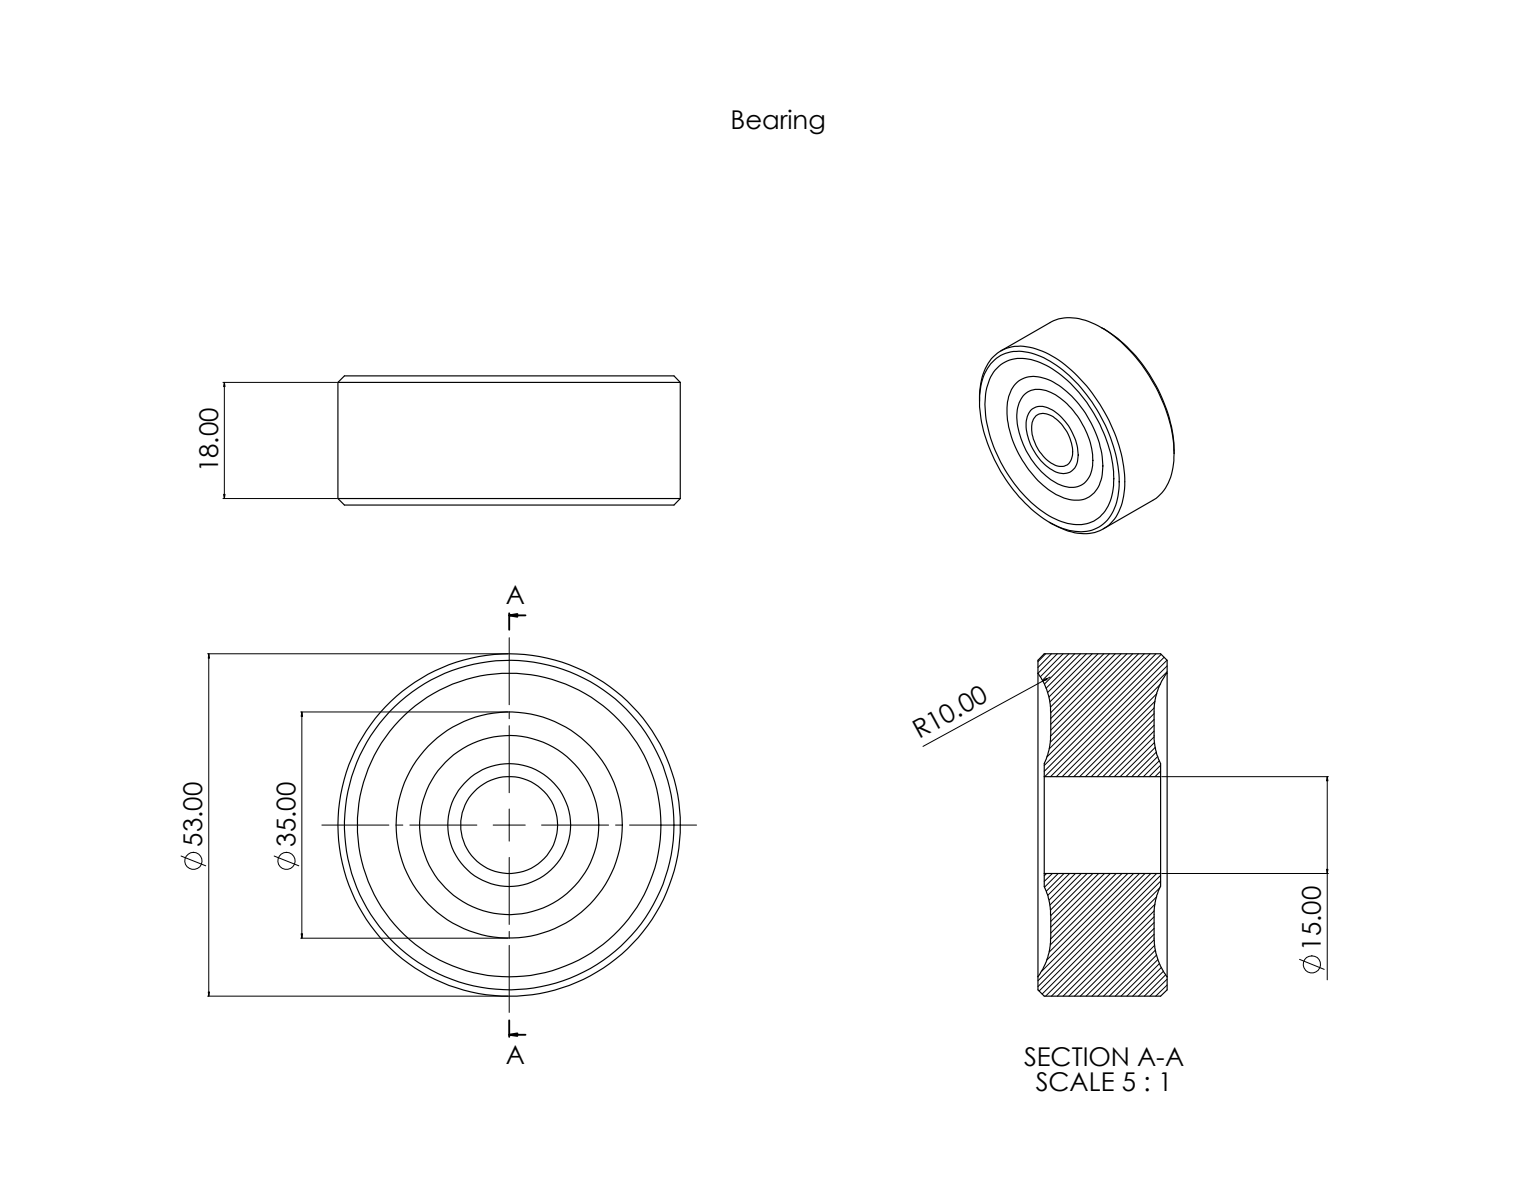
ISO-10303-21;
HEADER;
FILE_DESCRIPTION (('STEP AP214'),
    '1' );
FILE_NAME ('Bearing.step',
    '2026-10-19T17:36:30',
    ( '' ),
    ( '' ),
    'SwSTEP 2.0',
    'SolidWorks 2025',
    '' );
FILE_SCHEMA (( 'AUTOMOTIVE_DESIGN' ));
ENDSEC;

DATA;
#9=DIRECTION ( 'NONE',  ( -0.000000000000000000, -0.000000000000000000, -1.000000000000000000 ) ) ;
#14=DIRECTION ( 'NONE',  ( -0.000000000000000000, -0.000000000000000000, -1.000000000000000000 ) ) ;
#30=ORIENTED_EDGE ( 'NONE', *, *, #9025, .T. ) ;
#86=ADVANCED_FACE ( 'NONE', ( #9056 ), #3026, .F. ) ;
#151=CIRCLE ( 'NONE', #9264, 7.500000000000000000 ) ;
#175=EDGE_CURVE ( 'NONE', #10286, #4797, #4025, .T. ) ;
#182=DIRECTION ( 'NONE',  ( -0.7071067811865524577, 0.000000000000000000, -0.7071067811865426878 ) ) ;
#185=CONICAL_SURFACE ( 'NONE', #8085, 25.50000000000000711, 0.7853981633974552734 ) ;
#203=FACE_OUTER_BOUND ( 'NONE', #1468, .T. ) ;
#207=DIRECTION ( 'NONE',  ( 1.000000000000000000, 0.000000000000000000, 0.000000000000000000 ) ) ;
#209=DIRECTION ( 'NONE',  ( -0.000000000000000000, -0.000000000000000000, -1.000000000000000000 ) ) ;
#302=EDGE_CURVE ( 'NONE', #1347, #9626, #5867, .T. ) ;
#312=CIRCLE ( 'NONE', #4165, 9.499999999999994671 ) ;
#343=ADVANCED_FACE ( 'NONE', ( #7768 ), #9322, .F. ) ;
#362=( LENGTH_UNIT ( ) NAMED_UNIT ( * ) SI_UNIT ( .MILLI., .METRE. ) );
#374=CARTESIAN_POINT ( 'NONE',  ( 1.999999999999988010, 20.00000000000000355, 189.9999999999999716 ) ) ;
#386=DIRECTION ( 'NONE',  ( 0.000000000000000000, 0.000000000000000000, -1.000000000000000000 ) ) ;
#473=FACE_OUTER_BOUND ( 'NONE', #1842, .T. ) ;
#475=EDGE_CURVE ( 'NONE', #7179, #1407, #4444, .T. ) ;
#481=VERTEX_POINT ( 'NONE', #7503 ) ;
#524=DIRECTION ( 'NONE',  ( 1.000000000000000000, 0.000000000000000000, 0.000000000000000000 ) ) ;
#536=CARTESIAN_POINT ( 'NONE',  ( 27.49999999999999645, 20.00000000000000355, 189.9999999999999716 ) ) ;
#546=ADVANCED_FACE ( 'NONE', ( #3566 ), #11187, .T. ) ;
#568=CARTESIAN_POINT ( 'NONE',  ( 27.49999999999999645, 20.00000000000000355, 162.0000000000000000 ) ) ;
#631=DIRECTION ( 'NONE',  ( -0.000000000000000000, -0.000000000000000000, 1.000000000000000000 ) ) ;
#669=ORIENTED_EDGE ( 'NONE', *, *, #11328, .T. ) ;
#694=CARTESIAN_POINT ( 'NONE',  ( 27.49999999999999645, 20.00000000000000355, 189.9999999999999716 ) ) ;
#730=VERTEX_POINT ( 'NONE', #1726 ) ;
#754=DIRECTION ( 'NONE',  ( -0.000000000000000000, -0.000000000000000000, -1.000000000000000000 ) ) ;
#783=DIRECTION ( 'NONE',  ( 1.000000000000000000, 0.000000000000000000, 0.000000000000000000 ) ) ;
#792=ORIENTED_EDGE ( 'NONE', *, *, #1167, .F. ) ;
#818=CIRCLE ( 'NONE', #2648, 10.00000000000000000 ) ;
#833=EDGE_CURVE ( 'NONE', #4576, #10817, #6859, .T. ) ;
#847=EDGE_LOOP ( 'NONE', ( #1862, #12124, #11567, #792 ) ) ;
#851=CARTESIAN_POINT ( 'NONE',  ( 27.49999999999999645, 20.00000000000000355, 171.0000000000000000 ) ) ;
#856=CARTESIAN_POINT ( 'NONE',  ( 4.000000000000019540, 20.00000000000000711, 170.0000000000000000 ) ) ;
#861=DIRECTION ( 'NONE',  ( 1.000000000000000000, 0.000000000000000000, 0.000000000000000000 ) ) ;
#870=AXIS2_PLACEMENT_3D ( 'NONE', #1149, #3864, #4051 ) ;
#871=CARTESIAN_POINT ( 'NONE',  ( 1.000000000000000888, 20.00000000000000355, 170.9999999999999716 ) ) ;
#919=EDGE_CURVE ( 'NONE', #6911, #10286, #8230, .T. ) ;
#942=CARTESIAN_POINT ( 'NONE',  ( 41.35889894354065177, 20.00000000000000355, 162.0000000000000000 ) ) ;
#953=PRODUCT_CONTEXT ( 'NONE', #7801, 'mechanical' ) ;
#970=FACE_OUTER_BOUND ( 'NONE', #11386, .T. ) ;
#986=DIRECTION ( 'NONE',  ( 1.000000000000000000, 0.000000000000000000, 0.000000000000000000 ) ) ;
#998=DIRECTION ( 'NONE',  ( -0.000000000000000000, -0.000000000000000000, -1.000000000000000000 ) ) ;
#1040=FACE_OUTER_BOUND ( 'NONE', #4242, .T. ) ;
#1056=FACE_OUTER_BOUND ( 'NONE', #10210, .T. ) ;
#1061=ORIENTED_EDGE ( 'NONE', *, *, #10505, .T. ) ;
#1070=EDGE_CURVE ( 'NONE', #10817, #1347, #4044, .T. ) ;
#1075=AXIS2_PLACEMENT_3D ( 'NONE', #9726, #10725, #10926 ) ;
#1082=CIRCLE ( 'NONE', #11409, 17.49999999999996803 ) ;
#1094=AXIS2_PLACEMENT_3D ( 'NONE', #536, #2312, #8215 ) ;
#1097=CARTESIAN_POINT ( 'NONE',  ( 27.49999999999999645, 20.00000000000000355, 189.9999999999999716 ) ) ;
#1104=DIRECTION ( 'NONE',  ( 1.224646799147353207E-16, 1.000000000000000000, -0.000000000000000000 ) ) ;
#1122=CARTESIAN_POINT ( 'NONE',  ( 27.49999999999999645, 20.00000000000000355, 172.0000000000000000 ) ) ;
#1149=CARTESIAN_POINT ( 'NONE',  ( 27.49999999999999645, 20.00000000000000355, 189.9999999999999716 ) ) ;
#1157=FACE_OUTER_BOUND ( 'NONE', #5042, .T. ) ;
#1164=CARTESIAN_POINT ( 'NONE',  ( 19.99999999999999645, 20.00000000000000355, 189.9999999999999716 ) ) ;
#1167=EDGE_CURVE ( 'NONE', #1407, #9685, #1532, .T. ) ;
#1182=DIRECTION ( 'NONE',  ( 0.000000000000000000, 0.000000000000000000, -1.000000000000000000 ) ) ;
#1193=FACE_BOUND ( 'NONE', #3685, .T. ) ;
#1209=CARTESIAN_POINT ( 'NONE',  ( 27.49999999999999645, 20.00000000000000355, 189.9999999999999716 ) ) ;
#1211=AXIS2_PLACEMENT_3D ( 'NONE', #3932, #10461, #4763 ) ;
#1250=ORIENTED_EDGE ( 'NONE', *, *, #11960, .T. ) ;
#1305=CIRCLE ( 'NONE', #4943, 26.49999999999999645 ) ;
#1310=CARTESIAN_POINT ( 'NONE',  ( 27.49999999999999645, 20.00000000000000355, 170.0000000000000000 ) ) ;
#1318=AXIS2_PLACEMENT_3D ( 'NONE', #6837, #7793, #11665 ) ;
#1347=VERTEX_POINT ( 'NONE', #2706 ) ;
#1349=CARTESIAN_POINT ( 'NONE',  ( 27.49999999999999645, 20.00000000000000355, 197.9999999999999716 ) ) ;
#1369=AXIS2_PLACEMENT_3D ( 'NONE', #9446, #1818, #6703 ) ;
#1407=VERTEX_POINT ( 'NONE', #5698 ) ;
#1429=CARTESIAN_POINT ( 'NONE',  ( 34.99999999999999289, 20.00000000000000355, 171.0000000000000000 ) ) ;
#1446=TOROIDAL_SURFACE ( 'NONE', #12378, 13.85889894354065355, 10.00000000000000000 ) ;
#1468=EDGE_LOOP ( 'NONE', ( #3196, #7902 ) ) ;
#1499=AXIS2_PLACEMENT_3D ( 'NONE', #12513, #9480, #8642 ) ;
#1532=CIRCLE ( 'NONE', #6197, 10.00000000000000888 ) ;
#1544=ORIENTED_EDGE ( 'NONE', *, *, #11378, .T. ) ;
#1553=EDGE_CURVE ( 'NONE', #6911, #6345, #11267, .T. ) ;
#1584=AXIS2_PLACEMENT_3D ( 'NONE', #1209, #6901, #8873 ) ;
#1586=DIRECTION ( 'NONE',  ( 1.224646799147353207E-16, 1.000000000000000000, 0.000000000000000000 ) ) ;
#1598=EDGE_LOOP ( 'NONE', ( #3810, #5059 ) ) ;
#1620=DIRECTION ( 'NONE',  ( -0.000000000000000000, -0.000000000000000000, 1.000000000000000000 ) ) ;
#1675=PLANE ( 'NONE',  #2938 ) ;
#1700=CIRCLE ( 'NONE', #11843, 9.499999999999994671 ) ;
#1702=LINE ( 'NONE', #374, #11227 ) ;
#1726=CARTESIAN_POINT ( 'NONE',  ( 2.000000000000008882, 20.00000000000000711, 169.9999999999999716 ) ) ;
#1750=ORIENTED_EDGE ( 'NONE', *, *, #4293, .F. ) ;
#1791=EDGE_CURVE ( 'NONE', #8970, #4148, #8893, .T. ) ;
#1794=ORIENTED_EDGE ( 'NONE', *, *, #9260, .T. ) ;
#1818=DIRECTION ( 'NONE',  ( -0.000000000000000000, -0.000000000000000000, 1.000000000000000000 ) ) ;
#1821=FACE_OUTER_BOUND ( 'NONE', #2262, .T. ) ;
#1842=EDGE_LOOP ( 'NONE', ( #6785, #12387, #10361, #9801 ) ) ;
#1857=EDGE_CURVE ( 'NONE', #5215, #5293, #312, .T. ) ;
#1861=DIRECTION ( 'NONE',  ( 0.000000000000000000, 0.000000000000000000, -1.000000000000000000 ) ) ;
#1862=ORIENTED_EDGE ( 'NONE', *, *, #475, .F. ) ;
#1880=ADVANCED_FACE ( 'NONE', ( #8886, #203 ), #1675, .T. ) ;
#1893=AXIS2_PLACEMENT_3D ( 'NONE', #4279, #7320, #8219 ) ;
#1905=( NAMED_UNIT ( * ) SI_UNIT ( $, .STERADIAN. ) SOLID_ANGLE_UNIT ( ) );
#1926=DIRECTION ( 'NONE',  ( 0.000000000000000000, 0.000000000000000000, -1.000000000000000000 ) ) ;
#1928=VECTOR ( 'NONE', #3092, 1000.000000000000000 ) ;
#2003=TOROIDAL_SURFACE ( 'NONE', #3824, 13.85889894354065355, 10.00000000000000000 ) ;
#2075=AXIS2_PLACEMENT_3D ( 'NONE', #4841, #8707, #9787 ) ;
#2081=MANIFOLD_SOLID_BREP ( 'Fillet1', #9111 ) ;
#2093=DIRECTION ( 'NONE',  ( -0.000000000000000000, -0.000000000000000000, 1.000000000000000000 ) ) ;
#2098=DIRECTION ( 'NONE',  ( 1.000000000000000000, 0.000000000000000000, 0.000000000000000000 ) ) ;
#2107=CARTESIAN_POINT ( 'NONE',  ( 13.64110105645934290, 20.00000000000000355, 197.9999999999999716 ) ) ;
#2128=EDGE_LOOP ( 'NONE', ( #5597, #9875 ) ) ;
#2162=ORIENTED_EDGE ( 'NONE', *, *, #4585, .F. ) ;
#2167=DIRECTION ( 'NONE',  ( -0.000000000000000000, -0.000000000000000000, 1.000000000000000000 ) ) ;
#2177=VERTEX_POINT ( 'NONE', #10734 ) ;
#2208=CARTESIAN_POINT ( 'NONE',  ( 27.49999999999999645, 20.00000000000000355, 171.0000000000000000 ) ) ;
#2246=ORIENTED_EDGE ( 'NONE', *, *, #9611, .T. ) ;
#2262=EDGE_LOOP ( 'NONE', ( #5500, #669, #9036, #8194 ) ) ;
#2290=EDGE_LOOP ( 'NONE', ( #1544, #10095, #11839, #11489 ) ) ;
#2312=DIRECTION ( 'NONE',  ( 0.000000000000000000, 0.000000000000000000, -1.000000000000000000 ) ) ;
#2326=ORIENTED_EDGE ( 'NONE', *, *, #175, .F. ) ;
#2339=EDGE_LOOP ( 'NONE', ( #10440, #5022, #6178, #7639 ) ) ;
#2370=CARTESIAN_POINT ( 'NONE',  ( 18.00000000000000355, 20.00000000000000355, 171.0000000000000000 ) ) ;
#2372=DIRECTION ( 'NONE',  ( 1.000000000000000000, 0.000000000000000000, 0.000000000000000000 ) ) ;
#2373=CARTESIAN_POINT ( 'NONE',  ( 27.49999999999999645, 20.00000000000000355, 187.9999999999999716 ) ) ;
#2396=MECHANICAL_DESIGN_GEOMETRIC_PRESENTATION_REPRESENTATION('',(#6254),#7120);
#2404=FACE_BOUND ( 'NONE', #9472, .T. ) ;
#2443=AXIS2_PLACEMENT_3D ( 'NONE', #694, #12429, #4438 ) ;
#2520=AXIS2_PLACEMENT_3D ( 'NONE', #3090, #6958, #7856 ) ;
#2563=( NAMED_UNIT ( * ) SI_UNIT ( $, .STERADIAN. ) SOLID_ANGLE_UNIT ( ) );
#2576=ADVANCED_FACE ( 'NONE', ( #1157 ), #11345, .T. ) ;
#2634=AXIS2_PLACEMENT_3D ( 'NONE', #10717, #9844, #3935 ) ;
#2648=AXIS2_PLACEMENT_3D ( 'NONE', #9333, #1586, #12304 ) ;
#2706=CARTESIAN_POINT ( 'NONE',  ( 53.99999999999999289, 20.00000000000000711, 170.9999999999999716 ) ) ;
#2711=ORIENTED_EDGE ( 'NONE', *, *, #10237, .F. ) ;
#2715=CIRCLE ( 'NONE', #9816, 10.00000000000000888 ) ;
#2716=ADVANCED_FACE ( 'NONE', ( #4894 ), #4661, .F. ) ;
#2718=DIRECTION ( 'NONE',  ( 0.000000000000000000, 0.000000000000000000, -1.000000000000000000 ) ) ;
#2744=DIRECTION ( 'NONE',  ( 0.000000000000000000, 0.000000000000000000, 1.000000000000000000 ) ) ;
#2753=AXIS2_PLACEMENT_3D ( 'NONE', #11728, #3032, #12487 ) ;
#2782=ORIENTED_EDGE ( 'NONE', *, *, #7225, .T. ) ;
#2827=EDGE_LOOP ( 'NONE', ( #6882, #3164, #12009, #4594 ) ) ;
#2865=ADVANCED_FACE ( 'NONE', ( #7545, #5527 ), #4500, .T. ) ;
#2902=DIRECTION ( 'NONE',  ( -1.000000000000000000, 0.000000000000000000, 0.000000000000000000 ) ) ;
#2926=CIRCLE ( 'NONE', #2520, 25.50000000000000711 ) ;
#2933=DIRECTION ( 'NONE',  ( 0.000000000000000000, 0.000000000000000000, -1.000000000000000000 ) ) ;
#2935=( GEOMETRIC_REPRESENTATION_CONTEXT ( 3 ) GLOBAL_UNCERTAINTY_ASSIGNED_CONTEXT ( ( #3151 ) ) GLOBAL_UNIT_ASSIGNED_CONTEXT ( ( #10721, #5851, #1905 ) ) REPRESENTATION_CONTEXT ( 'NONE', 'WORKASPACE' ) );
#2938=AXIS2_PLACEMENT_3D ( 'NONE', #851, #1861, #7939 ) ;
#2959=DIRECTION ( 'NONE',  ( -1.000000000000000000, 0.000000000000000000, 0.000000000000000000 ) ) ;
#2965=DIRECTION ( 'NONE',  ( -0.000000000000000000, -0.000000000000000000, 1.000000000000000000 ) ) ;
#3005=ORIENTED_EDGE ( 'NONE', *, *, #10572, .T. ) ;
#3025=EDGE_CURVE ( 'NONE', #7179, #481, #818, .T. ) ;
#3026=TOROIDAL_SURFACE ( 'NONE', #6652, 17.49999999999996803, 10.00000000000000000 ) ;
#3032=DIRECTION ( 'NONE',  ( 0.000000000000000000, 0.000000000000000000, 1.000000000000000000 ) ) ;
#3070=CARTESIAN_POINT ( 'NONE',  ( 27.49999999999999645, 20.00000000000000355, 197.9999999999999716 ) ) ;
#3076=DIRECTION ( 'NONE',  ( -1.000000000000000000, 0.000000000000000000, 0.000000000000000000 ) ) ;
#3090=CARTESIAN_POINT ( 'NONE',  ( 27.49999999999999645, 20.00000000000000355, 189.9999999999999716 ) ) ;
#3092=DIRECTION ( 'NONE',  ( -0.000000000000000000, -0.000000000000000000, -1.000000000000000000 ) ) ;
#3100=CARTESIAN_POINT ( 'NONE',  ( 13.64110105645934290, 20.00000000000000355, 187.9999999999999716 ) ) ;
#3118=LINE ( 'NONE', #1164, #8438 ) ;
#3143=CARTESIAN_POINT ( 'NONE',  ( 27.49999999999999645, 20.00000000000000355, 172.0000000000000000 ) ) ;
#3151=UNCERTAINTY_MEASURE_WITH_UNIT (LENGTH_MEASURE( 1.000000000000000082E-05 ), #10721, 'distance_accuracy_value', 'NONE');
#3164=ORIENTED_EDGE ( 'NONE', *, *, #5095, .T. ) ;
#3168=AXIS2_PLACEMENT_3D ( 'NONE', #3277, #4032, #10889 ) ;
#3196=ORIENTED_EDGE ( 'NONE', *, *, #11378, .F. ) ;
#3201=CIRCLE ( 'NONE', #12514, 25.49999999999998934 ) ;
#3212=DIRECTION ( 'NONE',  ( -1.000000000000000000, 0.000000000000000000, 0.000000000000000000 ) ) ;
#3235=AXIS2_PLACEMENT_3D ( 'NONE', #3070, #11824, #2372 ) ;
#3253=ORIENTED_EDGE ( 'NONE', *, *, #9260, .F. ) ;
#3258=DIRECTION ( 'NONE',  ( -0.000000000000000000, -0.000000000000000000, -1.000000000000000000 ) ) ;
#3265=FACE_OUTER_BOUND ( 'NONE', #6855, .T. ) ;
#3277=CARTESIAN_POINT ( 'NONE',  ( 45.00000000000000000, 20.00000000000000711, 197.9999999999999716 ) ) ;
#3281=EDGE_CURVE ( 'NONE', #10732, #8970, #9129, .T. ) ;
#3299=ORIENTED_EDGE ( 'NONE', *, *, #9336, .F. ) ;
#3345=DIRECTION ( 'NONE',  ( 0.000000000000000000, 0.000000000000000000, -1.000000000000000000 ) ) ;
#3346=ADVANCED_FACE ( 'NONE', ( #6452, #4548 ), #7403, .F. ) ;
#3381=FACE_OUTER_BOUND ( 'NONE', #5742, .T. ) ;
#3411=AXIS2_PLACEMENT_3D ( 'NONE', #1122, #4987, #3076 ) ;
#3448=DIRECTION ( 'NONE',  ( 0.000000000000000000, 0.000000000000000000, 1.000000000000000000 ) ) ;
#3450=DIRECTION ( 'NONE',  ( 1.000000000000000000, 0.000000000000000000, 0.000000000000000000 ) ) ;
#3458=ORIENTED_EDGE ( 'NONE', *, *, #7225, .F. ) ;
#3485=ORIENTED_EDGE ( 'NONE', *, *, #833, .F. ) ;
#3519=DIRECTION ( 'NONE',  ( 0.000000000000000000, -1.000000000000000000, 0.000000000000000000 ) ) ;
#3563=EDGE_CURVE ( 'NONE', #730, #7703, #11363, .T. ) ;
#3566=FACE_OUTER_BOUND ( 'NONE', #7971, .T. ) ;
#3571=AXIS2_PLACEMENT_3D ( 'NONE', #1097, #209, #4425 ) ;
#3577=VERTEX_POINT ( 'NONE', #2370 ) ;
#3616=ORIENTED_EDGE ( 'NONE', *, *, #12033, .F. ) ;
#3620=EDGE_CURVE ( 'NONE', #10817, #4738, #11985, .T. ) ;
#3638=CARTESIAN_POINT ( 'NONE',  ( 27.49999999999999645, 20.00000000000000355, 188.9999999999999716 ) ) ;
#3664=CARTESIAN_POINT ( 'NONE',  ( 36.99999999999999289, 20.00000000000000355, 188.9999999999999716 ) ) ;
#3685=EDGE_LOOP ( 'NONE', ( #4549, #30 ) ) ;
#3712=VECTOR ( 'NONE', #10492, 1000.000000000000114 ) ;
#3721=TOROIDAL_SURFACE ( 'NONE', #10818, 17.49999999999996803, 10.00000000000000000 ) ;
#3723=DIRECTION ( 'NONE',  ( -1.000000000000000000, 0.000000000000000000, 0.000000000000000000 ) ) ;
#3749=VECTOR ( 'NONE', #11748, 1000.000000000000000 ) ;
#3752=DIRECTION ( 'NONE',  ( -0.000000000000000000, -0.000000000000000000, -1.000000000000000000 ) ) ;
#3774=CARTESIAN_POINT ( 'NONE',  ( 50.99999999999999289, 20.00000000000000711, 189.9999999999999716 ) ) ;
#3810=ORIENTED_EDGE ( 'NONE', *, *, #7903, .T. ) ;
#3814=AXIS2_PLACEMENT_3D ( 'NONE', #2107, #1104, #5984 ) ;
#3824=AXIS2_PLACEMENT_3D ( 'NONE', #9746, #10883, #7840 ) ;
#3851=DIRECTION ( 'NONE',  ( -1.000000000000000000, 0.000000000000000000, 0.000000000000000000 ) ) ;
#3864=DIRECTION ( 'NONE',  ( 0.000000000000000000, 0.000000000000000000, 1.000000000000000000 ) ) ;
#3901=ORIENTED_EDGE ( 'NONE', *, *, #3563, .F. ) ;
#3917=PLANE ( 'NONE',  #1318 ) ;
#3923=ADVANCED_FACE ( 'NONE', ( #6163 ), #1446, .F. ) ;
#3932=CARTESIAN_POINT ( 'NONE',  ( 27.49999999999999645, 20.00000000000000355, 187.9999999999999716 ) ) ;
#3935=DIRECTION ( 'NONE',  ( 1.000000000000000000, 0.000000000000000000, 0.000000000000000000 ) ) ;
#3940=SHAPE_REPRESENTATION_RELATIONSHIP ( 'NONE' , 'NONE' ,  #10013, #4901 ) ;
#3958=DIRECTION ( 'NONE',  ( 0.000000000000000000, 0.000000000000000000, -1.000000000000000000 ) ) ;
#4025=CIRCLE ( 'NONE', #7680, 10.00000000000000888 ) ;
#4032=DIRECTION ( 'NONE',  ( -1.224646799147353207E-16, 1.000000000000000000, 0.000000000000000000 ) ) ;
#4044=LINE ( 'NONE', #9955, #1928 ) ;
#4051=DIRECTION ( 'NONE',  ( 1.000000000000000000, 0.000000000000000000, 0.000000000000000000 ) ) ;
#4142=AXIS2_PLACEMENT_3D ( 'NONE', #9560, #12533, #861 ) ;
#4148=VERTEX_POINT ( 'NONE', #8436 ) ;
#4164=EDGE_LOOP ( 'NONE', ( #1794, #4301 ) ) ;
#4165=AXIS2_PLACEMENT_3D ( 'NONE', #3638, #6617, #9845 ) ;
#4225=CIRCLE ( 'NONE', #1584, 25.50000000000000711 ) ;
#4242=EDGE_LOOP ( 'NONE', ( #1061, #9593, #2711, #3299 ) ) ;
#4279=CARTESIAN_POINT ( 'NONE',  ( 27.49999999999999645, 20.00000000000000355, 188.9999999999999716 ) ) ;
#4288=ORIENTED_EDGE ( 'NONE', *, *, #7758, .T. ) ;
#4293=EDGE_CURVE ( 'NONE', #4576, #2177, #4225, .T. ) ;
#4301=ORIENTED_EDGE ( 'NONE', *, *, #3563, .T. ) ;
#4316=DIRECTION ( 'NONE',  ( 0.000000000000000000, 0.000000000000000000, 1.000000000000000000 ) ) ;
#4341=VECTOR ( 'NONE', #3752, 1000.000000000000000 ) ;
#4374=DIRECTION ( 'NONE',  ( 1.000000000000000000, 0.000000000000000000, 0.000000000000000000 ) ) ;
#4410=AXIS2_PLACEMENT_3D ( 'NONE', #2373, #10940, #3450 ) ;
#4425=DIRECTION ( 'NONE',  ( -1.000000000000000000, 0.000000000000000000, 0.000000000000000000 ) ) ;
#4438=DIRECTION ( 'NONE',  ( 1.000000000000000000, 0.000000000000000000, -0.000000000000000000 ) ) ;
#4439=ORIENTED_EDGE ( 'NONE', *, *, #10182, .F. ) ;
#4444=CIRCLE ( 'NONE', #7080, 23.49999999999999289 ) ;
#4500=PLANE ( 'NONE',  #2443 ) ;
#4548=FACE_BOUND ( 'NONE', #2128, .T. ) ;
#4549=ORIENTED_EDGE ( 'NONE', *, *, #7622, .T. ) ;
#4558=CARTESIAN_POINT ( 'NONE',  ( 18.00000000000000355, 20.00000000000000355, 188.9999999999999716 ) ) ;
#4576=VERTEX_POINT ( 'NONE', #8787 ) ;
#4585=EDGE_CURVE ( 'NONE', #11119, #10746, #6848, .T. ) ;
#4587=DIRECTION ( 'NONE',  ( 0.000000000000000000, -1.000000000000000000, 0.000000000000000000 ) ) ;
#4594=ORIENTED_EDGE ( 'NONE', *, *, #7758, .F. ) ;
#4610=DIRECTION ( 'NONE',  ( 0.000000000000000000, 0.000000000000000000, 1.000000000000000000 ) ) ;
#4661=TOROIDAL_SURFACE ( 'NONE', #9531, 17.50000000000000355, 10.00000000000000000 ) ;
#4689=ORIENTED_EDGE ( 'NONE', *, *, #5994, .F. ) ;
#4723=DIRECTION ( 'NONE',  ( -0.000000000000000000, -0.000000000000000000, 1.000000000000000000 ) ) ;
#4738=VERTEX_POINT ( 'NONE', #10183 ) ;
#4763=DIRECTION ( 'NONE',  ( 1.000000000000000000, 0.000000000000000000, 0.000000000000000000 ) ) ;
#4797=VERTEX_POINT ( 'NONE', #8157 ) ;
#4806=CIRCLE ( 'NONE', #8050, 7.500000000000000000 ) ;
#4820=CONICAL_SURFACE ( 'NONE', #6439, 26.49999999999999645, 0.7853981633974517207 ) ;
#4833=CARTESIAN_POINT ( 'NONE',  ( 27.49999999999999645, 20.00000000000000355, 197.9999999999999716 ) ) ;
#4841=CARTESIAN_POINT ( 'NONE',  ( 27.49999999999999645, 20.00000000000000355, 172.0000000000000000 ) ) ;
#4868=ORIENTED_EDGE ( 'NONE', *, *, #1553, .T. ) ;
#4894=FACE_OUTER_BOUND ( 'NONE', #6222, .T. ) ;
#4901=ADVANCED_BREP_SHAPE_REPRESENTATION ( '', ( #2081, #9021 ), #2935 ) ;
#4918=DIRECTION ( 'NONE',  ( -1.000000000000000000, 0.000000000000000000, 0.000000000000000000 ) ) ;
#4943=AXIS2_PLACEMENT_3D ( 'NONE', #12527, #1926, #11578 ) ;
#4987=DIRECTION ( 'NONE',  ( -0.000000000000000000, -0.000000000000000000, 1.000000000000000000 ) ) ;
#4988=ORIENTED_EDGE ( 'NONE', *, *, #9025, .F. ) ;
#4995=ORIENTED_EDGE ( 'NONE', *, *, #4585, .T. ) ;
#5022=ORIENTED_EDGE ( 'NONE', *, *, #919, .T. ) ;
#5042=EDGE_LOOP ( 'NONE', ( #9489, #3253, #2782, #7875 ) ) ;
#5059=ORIENTED_EDGE ( 'NONE', *, *, #1857, .T. ) ;
#5073=DIRECTION ( 'NONE',  ( -0.000000000000000000, -0.000000000000000000, -1.000000000000000000 ) ) ;
#5095=EDGE_CURVE ( 'NONE', #5215, #8335, #9299, .T. ) ;
#5179=DIRECTION ( 'NONE',  ( -0.000000000000000000, -0.000000000000000000, 1.000000000000000000 ) ) ;
#5187=EDGE_LOOP ( 'NONE', ( #5513, #6283 ) ) ;
#5215=VERTEX_POINT ( 'NONE', #4558 ) ;
#5245=ADVANCED_FACE ( 'NONE', ( #12301 ), #185, .T. ) ;
#5258=CIRCLE ( 'NONE', #1211, 17.50000000000000000 ) ;
#5259=CARTESIAN_POINT ( 'NONE',  ( 34.99999999999999289, 20.00000000000000355, 189.9999999999999716 ) ) ;
#5261=AXIS2_PLACEMENT_3D ( 'NONE', #5821, #4723, #986 ) ;
#5293=VERTEX_POINT ( 'NONE', #3664 ) ;
#5332=CIRCLE ( 'NONE', #1075, 9.499999999999994671 ) ;
#5349=CIRCLE ( 'NONE', #1499, 13.85889894354065710 ) ;
#5373=CIRCLE ( 'NONE', #4142, 26.49999999999999645 ) ;
#5420=DIRECTION ( 'NONE',  ( -0.000000000000000000, -0.000000000000000000, 1.000000000000000000 ) ) ;
#5451=AXIS2_PLACEMENT_3D ( 'NONE', #6681, #2093, #11803 ) ;
#5499=AXIS2_PLACEMENT_3D ( 'NONE', #6392, #4610, #5572 ) ;
#5500=ORIENTED_EDGE ( 'NONE', *, *, #3281, .F. ) ;
#5513=ORIENTED_EDGE ( 'NONE', *, *, #12033, .T. ) ;
#5523=CARTESIAN_POINT ( 'NONE',  ( 45.00000000000000000, 20.00000000000000711, 187.9999999999999716 ) ) ;
#5527=FACE_BOUND ( 'NONE', #5645, .T. ) ;
#5572=DIRECTION ( 'NONE',  ( 1.000000000000000000, 0.000000000000000000, -0.000000000000000000 ) ) ;
#5580=DIRECTION ( 'NONE',  ( -1.000000000000000000, 0.000000000000000000, 0.000000000000000000 ) ) ;
#5597=ORIENTED_EDGE ( 'NONE', *, *, #5994, .T. ) ;
#5633=CARTESIAN_POINT ( 'NONE',  ( 27.49999999999999645, 20.00000000000000355, 172.0000000000000000 ) ) ;
#5645=EDGE_LOOP ( 'NONE', ( #8468, #9144 ) ) ;
#5698=CARTESIAN_POINT ( 'NONE',  ( 50.99999999999997868, 20.00000000000000355, 170.0000000000000000 ) ) ;
#5705=CARTESIAN_POINT ( 'NONE',  ( 34.99999999999999289, 20.00000000000000355, 188.9999999999999716 ) ) ;
#5742=EDGE_LOOP ( 'NONE', ( #7247, #11998 ) ) ;
#5782=ORIENTED_EDGE ( 'NONE', *, *, #7927, .F. ) ;
#5816=VERTEX_POINT ( 'NONE', #7526 ) ;
#5821=CARTESIAN_POINT ( 'NONE',  ( 27.49999999999999645, 20.00000000000000355, 170.9999999999999716 ) ) ;
#5835=SHAPE_DEFINITION_REPRESENTATION ( #10056, #10013 ) ;
#5839=ADVANCED_FACE ( 'NONE', ( #7713 ), #2003, .F. ) ;
#5851=( NAMED_UNIT ( * ) PLANE_ANGLE_UNIT ( ) SI_UNIT ( $, .RADIAN. ) );
#5867=CIRCLE ( 'NONE', #5261, 26.49999999999999645 ) ;
#5897=AXIS2_PLACEMENT_3D ( 'NONE', #8209, #3258, #11061 ) ;
#5942=EDGE_LOOP ( 'NONE', ( #11633, #8084, #4288, #4988 ) ) ;
#5984=DIRECTION ( 'NONE',  ( -1.000000000000000000, 0.000000000000000000, 0.000000000000000000 ) ) ;
#5994=EDGE_CURVE ( 'NONE', #1407, #7179, #9107, .T. ) ;
#6077=EDGE_CURVE ( 'NONE', #4797, #6345, #5258, .T. ) ;
#6132=ORIENTED_EDGE ( 'NONE', *, *, #1167, .T. ) ;
#6163=FACE_OUTER_BOUND ( 'NONE', #5942, .T. ) ;
#6165=AXIS2_PLACEMENT_3D ( 'NONE', #8779, #1182, #4918 ) ;
#6173=AXIS2_PLACEMENT_3D ( 'NONE', #7250, #3448, #7313 ) ;
#6178=ORIENTED_EDGE ( 'NONE', *, *, #175, .T. ) ;
#6197=AXIS2_PLACEMENT_3D ( 'NONE', #11340, #11273, #3345 ) ;
#6222=EDGE_LOOP ( 'NONE', ( #11236, #4868, #6358, #2326 ) ) ;
#6233=CIRCLE ( 'NONE', #4410, 13.85889894354065710 ) ;
#6254=STYLED_ITEM('',(#12584),#2081);
#6280=CARTESIAN_POINT ( 'NONE',  ( 27.49999999999999645, 20.00000000000000355, 172.0000000000000000 ) ) ;
#6283=ORIENTED_EDGE ( 'NONE', *, *, #4293, .T. ) ;
#6309=CARTESIAN_POINT ( 'NONE',  ( 27.49999999999999645, 20.00000000000000355, 189.9999999999999716 ) ) ;
#6321=DIRECTION ( 'NONE',  ( 1.000000000000000000, 0.000000000000000000, 0.000000000000000000 ) ) ;
#6341=FACE_OUTER_BOUND ( 'NONE', #847, .T. ) ;
#6345=VERTEX_POINT ( 'NONE', #5523 ) ;
#6358=ORIENTED_EDGE ( 'NONE', *, *, #6077, .F. ) ;
#6392=CARTESIAN_POINT ( 'NONE',  ( 27.49999999999999645, 20.00000000000000355, 169.9999999999999716 ) ) ;
#6439=AXIS2_PLACEMENT_3D ( 'NONE', #7693, #2167, #2098 ) ;
#6452=FACE_OUTER_BOUND ( 'NONE', #4164, .T. ) ;
#6485=CARTESIAN_POINT ( 'NONE',  ( 27.49999999999999645, 20.00000000000000355, 170.0000000000000000 ) ) ;
#6502=CARTESIAN_POINT ( 'NONE',  ( 53.99999999999999289, 20.00000000000000355, 170.9999999999999716 ) ) ;
#6551=AXIS2_PLACEMENT_3D ( 'NONE', #9813, #998, #3212 ) ;
#6610=CIRCLE ( 'NONE', #12096, 13.85889894354065355 ) ;
#6617=DIRECTION ( 'NONE',  ( 0.000000000000000000, 0.000000000000000000, 1.000000000000000000 ) ) ;
#6652=AXIS2_PLACEMENT_3D ( 'NONE', #9491, #1620, #6321 ) ;
#6681=CARTESIAN_POINT ( 'NONE',  ( 27.49999999999999645, 20.00000000000000355, 171.0000000000000000 ) ) ;
#6703=DIRECTION ( 'NONE',  ( 1.000000000000000000, 0.000000000000000000, 0.000000000000000000 ) ) ;
#6785=ORIENTED_EDGE ( 'NONE', *, *, #1070, .F. ) ;
#6792=ORIENTED_EDGE ( 'NONE', *, *, #8850, .T. ) ;
#6833=DIRECTION ( 'NONE',  ( -0.000000000000000000, -0.000000000000000000, 1.000000000000000000 ) ) ;
#6837=CARTESIAN_POINT ( 'NONE',  ( 27.49999999999999645, 20.00000000000000355, 188.9999999999999716 ) ) ;
#6848=CIRCLE ( 'NONE', #3411, 13.85889894354065355 ) ;
#6855=EDGE_LOOP ( 'NONE', ( #1750, #10407, #8775, #9220 ) ) ;
#6859=LINE ( 'NONE', #8958, #3749 ) ;
#6882=ORIENTED_EDGE ( 'NONE', *, *, #1857, .F. ) ;
#6901=DIRECTION ( 'NONE',  ( 0.000000000000000000, 0.000000000000000000, 1.000000000000000000 ) ) ;
#6911=VERTEX_POINT ( 'NONE', #3774 ) ;
#6918=DIRECTION ( 'NONE',  ( 1.000000000000000000, 0.000000000000000000, 0.000000000000000000 ) ) ;
#6958=DIRECTION ( 'NONE',  ( 0.000000000000000000, 0.000000000000000000, 1.000000000000000000 ) ) ;
#6986=CARTESIAN_POINT ( 'NONE',  ( 27.49999999999999645, 20.00000000000000355, 169.9999999999999716 ) ) ;
#6994=ADVANCED_FACE ( 'NONE', ( #8728 ), #12034, .F. ) ;
#6998=EDGE_CURVE ( 'NONE', #9685, #481, #1082, .T. ) ;
#7080=AXIS2_PLACEMENT_3D ( 'NONE', #6485, #5420, #9291 ) ;
#7120=( GEOMETRIC_REPRESENTATION_CONTEXT ( 3 ) GLOBAL_UNCERTAINTY_ASSIGNED_CONTEXT ( ( #11655 ) ) GLOBAL_UNIT_ASSIGNED_CONTEXT ( ( #362, #12213, #2563 ) ) REPRESENTATION_CONTEXT ( 'NONE', 'WORKASPACE' ) );
#7153=EDGE_CURVE ( 'NONE', #4738, #10817, #1305, .T. ) ;
#7160=FACE_OUTER_BOUND ( 'NONE', #12382, .T. ) ;
#7164=ORIENTED_EDGE ( 'NONE', *, *, #7927, .T. ) ;
#7179=VERTEX_POINT ( 'NONE', #856 ) ;
#7225=EDGE_CURVE ( 'NONE', #7703, #1347, #12345, .T. ) ;
#7247=ORIENTED_EDGE ( 'NONE', *, *, #6077, .T. ) ;
#7248=CARTESIAN_POINT ( 'NONE',  ( 27.49999999999999645, 20.00000000000000355, 189.0000000000000000 ) ) ;
#7250=CARTESIAN_POINT ( 'NONE',  ( 27.49999999999999645, 20.00000000000000355, 187.9999999999999716 ) ) ;
#7251=DIRECTION ( 'NONE',  ( -1.000000000000000000, 0.000000000000000000, 0.000000000000000000 ) ) ;
#7303=ADVANCED_FACE ( 'NONE', ( #1056 ), #9199, .F. ) ;
#7313=DIRECTION ( 'NONE',  ( 1.000000000000000000, 0.000000000000000000, -0.000000000000000000 ) ) ;
#7320=DIRECTION ( 'NONE',  ( 0.000000000000000000, 0.000000000000000000, 1.000000000000000000 ) ) ;
#7395=CARTESIAN_POINT ( 'NONE',  ( 13.64110105645934290, 20.00000000000000355, 162.0000000000000000 ) ) ;
#7403=PLANE ( 'NONE',  #5499 ) ;
#7440=DIRECTION ( 'NONE',  ( -0.000000000000000000, -0.000000000000000000, -1.000000000000000000 ) ) ;
#7472=DIRECTION ( 'NONE',  ( -1.224646799147353207E-16, 1.000000000000000000, 0.000000000000000000 ) ) ;
#7495=EDGE_LOOP ( 'NONE', ( #8435, #9099 ) ) ;
#7503=CARTESIAN_POINT ( 'NONE',  ( 10.00000000000003020, 20.00000000000000711, 172.0000000000000000 ) ) ;
#7525=CARTESIAN_POINT ( 'NONE',  ( 41.35889894354065177, 20.00000000000000355, 187.9999999999999716 ) ) ;
#7526=CARTESIAN_POINT ( 'NONE',  ( 19.99999999999999645, 20.00000000000000355, 188.9999999999999716 ) ) ;
#7544=ADVANCED_FACE ( 'NONE', ( #3265 ), #9805, .T. ) ;
#7545=FACE_OUTER_BOUND ( 'NONE', #5187, .T. ) ;
#7561=EDGE_LOOP ( 'NONE', ( #7625, #7788 ) ) ;
#7586=CIRCLE ( 'NONE', #1893, 7.500000000000000000 ) ;
#7601=AXIS2_PLACEMENT_3D ( 'NONE', #7395, #10541, #2933 ) ;
#7622=EDGE_CURVE ( 'NONE', #10986, #8335, #5349, .T. ) ;
#7625=ORIENTED_EDGE ( 'NONE', *, *, #10505, .F. ) ;
#7639=ORIENTED_EDGE ( 'NONE', *, *, #10029, .F. ) ;
#7680=AXIS2_PLACEMENT_3D ( 'NONE', #12217, #3519, #3958 ) ;
#7693=CARTESIAN_POINT ( 'NONE',  ( 27.49999999999999645, 20.00000000000000355, 170.9999999999999716 ) ) ;
#7696=DIRECTION ( 'NONE',  ( 0.000000000000000000, 0.000000000000000000, 1.000000000000000000 ) ) ;
#7703=VERTEX_POINT ( 'NONE', #10540 ) ;
#7713=FACE_OUTER_BOUND ( 'NONE', #2290, .T. ) ;
#7728=EDGE_CURVE ( 'NONE', #4738, #9626, #8581, .T. ) ;
#7732=CARTESIAN_POINT ( 'NONE',  ( 27.49999999999999645, 20.00000000000000355, 189.9999999999999716 ) ) ;
#7758=EDGE_CURVE ( 'NONE', #5293, #10986, #2715, .T. ) ;
#7768=FACE_OUTER_BOUND ( 'NONE', #2827, .T. ) ;
#7769=LINE ( 'NONE', #9740, #7853 ) ;
#7787=AXIS2_PLACEMENT_3D ( 'NONE', #7732, #754, #3723 ) ;
#7788=ORIENTED_EDGE ( 'NONE', *, *, #11328, .F. ) ;
#7793=DIRECTION ( 'NONE',  ( 0.000000000000000000, 0.000000000000000000, 1.000000000000000000 ) ) ;
#7801=APPLICATION_CONTEXT ( 'automotive_design' ) ;
#7821=CARTESIAN_POINT ( 'NONE',  ( 27.49999999999999645, 20.00000000000000355, 188.9999999999999716 ) ) ;
#7840=DIRECTION ( 'NONE',  ( -1.000000000000000000, 0.000000000000000000, 0.000000000000000000 ) ) ;
#7848=AXIS2_PLACEMENT_3D ( 'NONE', #942, #7472, #3851 ) ;
#7853=VECTOR ( 'NONE', #11641, 1000.000000000000114 ) ;
#7856=DIRECTION ( 'NONE',  ( 1.000000000000000000, 0.000000000000000000, 0.000000000000000000 ) ) ;
#7875=ORIENTED_EDGE ( 'NONE', *, *, #12257, .F. ) ;
#7902=ORIENTED_EDGE ( 'NONE', *, *, #10132, .F. ) ;
#7903=EDGE_CURVE ( 'NONE', #5293, #5215, #5332, .T. ) ;
#7927=EDGE_CURVE ( 'NONE', #481, #9685, #11607, .T. ) ;
#7939=DIRECTION ( 'NONE',  ( 1.000000000000000000, 0.000000000000000000, 0.000000000000000000 ) ) ;
#7971=EDGE_LOOP ( 'NONE', ( #11116, #10735, #8923, #9671 ) ) ;
#8021=ORIENTED_EDGE ( 'NONE', *, *, #3620, .F. ) ;
#8050=AXIS2_PLACEMENT_3D ( 'NONE', #7821, #7696, #8643 ) ;
#8052=APPLICATION_CONTEXT ( 'automotive_design' ) ;
#8084=ORIENTED_EDGE ( 'NONE', *, *, #7903, .F. ) ;
#8085=AXIS2_PLACEMENT_3D ( 'NONE', #8679, #2718, #5580 ) ;
#8105=AXIS2_PLACEMENT_3D ( 'NONE', #9355, #7440, #7251 ) ;
#8148=DIRECTION ( 'NONE',  ( 0.000000000000000000, 0.000000000000000000, -1.000000000000000000 ) ) ;
#8157=CARTESIAN_POINT ( 'NONE',  ( 9.999999999999991118, 20.00000000000000355, 187.9999999999999716 ) ) ;
#8194=ORIENTED_EDGE ( 'NONE', *, *, #1791, .F. ) ;
#8209=CARTESIAN_POINT ( 'NONE',  ( 27.49999999999999645, 20.00000000000000355, 169.9999999999999716 ) ) ;
#8214=CIRCLE ( 'NONE', #7601, 10.00000000000000888 ) ;
#8215=DIRECTION ( 'NONE',  ( -1.000000000000000000, 0.000000000000000000, 0.000000000000000000 ) ) ;
#8219=DIRECTION ( 'NONE',  ( 1.000000000000000000, 0.000000000000000000, 0.000000000000000000 ) ) ;
#8230=CIRCLE ( 'NONE', #2753, 23.49999999999999289 ) ;
#8303=ORIENTED_EDGE ( 'NONE', *, *, #6998, .T. ) ;
#8321=EDGE_CURVE ( 'NONE', #10286, #6911, #10388, .T. ) ;
#8335=VERTEX_POINT ( 'NONE', #3100 ) ;
#8415=ADVANCED_FACE ( 'NONE', ( #7160, #2404 ), #9202, .T. ) ;
#8426=DIRECTION ( 'NONE',  ( 0.000000000000000000, 0.000000000000000000, 1.000000000000000000 ) ) ;
#8435=ORIENTED_EDGE ( 'NONE', *, *, #10237, .T. ) ;
#8436=CARTESIAN_POINT ( 'NONE',  ( 19.99999999999999645, 20.00000000000000355, 171.0000000000000000 ) ) ;
#8438=VECTOR ( 'NONE', #14, 1000.000000000000000 ) ;
#8468=ORIENTED_EDGE ( 'NONE', *, *, #8321, .F. ) ;
#8517=VECTOR ( 'NONE', #5073, 1000.000000000000000 ) ;
#8581=LINE ( 'NONE', #9542, #4341 ) ;
#8642=DIRECTION ( 'NONE',  ( 1.000000000000000000, 0.000000000000000000, 0.000000000000000000 ) ) ;
#8643=DIRECTION ( 'NONE',  ( 1.000000000000000000, 0.000000000000000000, 0.000000000000000000 ) ) ;
#8679=CARTESIAN_POINT ( 'NONE',  ( 27.49999999999999645, 20.00000000000000355, 189.9999999999999716 ) ) ;
#8688=AXIS2_PLACEMENT_3D ( 'NONE', #1310, #5179, #524 ) ;
#8707=DIRECTION ( 'NONE',  ( 0.000000000000000000, 0.000000000000000000, -1.000000000000000000 ) ) ;
#8728=FACE_OUTER_BOUND ( 'NONE', #2339, .T. ) ;
#8740=FACE_BOUND ( 'NONE', #7561, .T. ) ;
#8755=DIRECTION ( 'NONE',  ( -1.000000000000000000, 0.000000000000000000, 0.000000000000000000 ) ) ;
#8775=ORIENTED_EDGE ( 'NONE', *, *, #7153, .F. ) ;
#8779=CARTESIAN_POINT ( 'NONE',  ( 27.49999999999999645, 20.00000000000000355, 162.0000000000000000 ) ) ;
#8787=CARTESIAN_POINT ( 'NONE',  ( 53.00000000000000711, 20.00000000000000711, 189.9999999999999716 ) ) ;
#8788=EDGE_LOOP ( 'NONE', ( #11491, #4689, #6132, #5782 ) ) ;
#8850=EDGE_CURVE ( 'NONE', #730, #9626, #7769, .T. ) ;
#8873=DIRECTION ( 'NONE',  ( 1.000000000000000000, 0.000000000000000000, 0.000000000000000000 ) ) ;
#8886=FACE_BOUND ( 'NONE', #7495, .T. ) ;
#8893=CIRCLE ( 'NONE', #5451, 7.500000000000000000 ) ;
#8915=ORIENTED_EDGE ( 'NONE', *, *, #10132, .T. ) ;
#8923=ORIENTED_EDGE ( 'NONE', *, *, #302, .T. ) ;
#8958=CARTESIAN_POINT ( 'NONE',  ( 53.00000000000000711, 20.00000000000000711, 189.9999999999999716 ) ) ;
#8970=VERTEX_POINT ( 'NONE', #1429 ) ;
#8974=ADVANCED_FACE ( 'NONE', ( #473 ), #11188, .T. ) ;
#9021=AXIS2_PLACEMENT_3D ( 'NONE', #11433, #2744, #207 ) ;
#9025=EDGE_CURVE ( 'NONE', #8335, #10986, #6233, .T. ) ;
#9036=ORIENTED_EDGE ( 'NONE', *, *, #9336, .T. ) ;
#9056=FACE_OUTER_BOUND ( 'NONE', #8788, .T. ) ;
#9099=ORIENTED_EDGE ( 'NONE', *, *, #1791, .T. ) ;
#9107=CIRCLE ( 'NONE', #8688, 23.49999999999999289 ) ;
#9111=CLOSED_SHELL ( 'NONE', ( #2716, #343, #5839, #11720, #7544, #9315, #546, #9382, #12380, #11846, #2865, #3346, #8974, #8415, #2576, #5245, #11947, #1880, #86, #7303, #3923, #6994 ) ) ;
#9129=LINE ( 'NONE', #5259, #8517 ) ;
#9144=ORIENTED_EDGE ( 'NONE', *, *, #919, .F. ) ;
#9145=AXIS2_PLACEMENT_3D ( 'NONE', #7248, #8148, #11121 ) ;
#9159=VERTEX_POINT ( 'NONE', #11246 ) ;
#9199=TOROIDAL_SURFACE ( 'NONE', #6165, 13.85889894354065355, 10.00000000000000000 ) ;
#9202=PLANE ( 'NONE',  #10583 ) ;
#9220=ORIENTED_EDGE ( 'NONE', *, *, #11960, .F. ) ;
#9230=DIRECTION ( 'NONE',  ( -0.000000000000000000, -0.000000000000000000, -1.000000000000000000 ) ) ;
#9260=EDGE_CURVE ( 'NONE', #7703, #730, #3201, .T. ) ;
#9264=AXIS2_PLACEMENT_3D ( 'NONE', #2208, #6833, #10822 ) ;
#9274=CIRCLE ( 'NONE', #7848, 10.00000000000000178 ) ;
#9291=DIRECTION ( 'NONE',  ( 1.000000000000000000, 0.000000000000000000, 0.000000000000000000 ) ) ;
#9299=CIRCLE ( 'NONE', #3814, 10.00000000000000000 ) ;
#9315=ADVANCED_FACE ( 'NONE', ( #970 ), #4820, .T. ) ;
#9322=TOROIDAL_SURFACE ( 'NONE', #3235, 13.85889894354065355, 10.00000000000000000 ) ;
#9333=CARTESIAN_POINT ( 'NONE',  ( 10.00000000000003020, 20.00000000000000711, 162.0000000000000000 ) ) ;
#9336=EDGE_CURVE ( 'NONE', #5816, #4148, #3118, .T. ) ;
#9355=CARTESIAN_POINT ( 'NONE',  ( 27.49999999999999645, 20.00000000000000355, 189.9999999999999716 ) ) ;
#9382=ADVANCED_FACE ( 'NONE', ( #1040 ), #11687, .F. ) ;
#9418=CARTESIAN_POINT ( 'NONE',  ( 41.35889894354065177, 20.00000000000000355, 197.9999999999999716 ) ) ;
#9446=CARTESIAN_POINT ( 'NONE',  ( 27.49999999999999645, 20.00000000000000355, 171.0000000000000000 ) ) ;
#9460=CIRCLE ( 'NONE', #11898, 17.50000000000000000 ) ;
#9472=EDGE_LOOP ( 'NONE', ( #2246, #4995 ) ) ;
#9480=DIRECTION ( 'NONE',  ( -0.000000000000000000, -0.000000000000000000, -1.000000000000000000 ) ) ;
#9489=ORIENTED_EDGE ( 'NONE', *, *, #8850, .F. ) ;
#9491=CARTESIAN_POINT ( 'NONE',  ( 27.49999999999999645, 20.00000000000000355, 162.0000000000000000 ) ) ;
#9531=AXIS2_PLACEMENT_3D ( 'NONE', #4833, #9, #8755 ) ;
#9542=CARTESIAN_POINT ( 'NONE',  ( 1.000000000000000888, 20.00000000000000355, 189.9999999999999716 ) ) ;
#9560=CARTESIAN_POINT ( 'NONE',  ( 27.49999999999999645, 20.00000000000000355, 170.9999999999999716 ) ) ;
#9573=FACE_OUTER_BOUND ( 'NONE', #1598, .T. ) ;
#9593=ORIENTED_EDGE ( 'NONE', *, *, #3281, .T. ) ;
#9611=EDGE_CURVE ( 'NONE', #10746, #11119, #6610, .T. ) ;
#9626=VERTEX_POINT ( 'NONE', #871 ) ;
#9634=CARTESIAN_POINT ( 'NONE',  ( 13.64110105645934290, 20.00000000000000355, 172.0000000000000000 ) ) ;
#9671=ORIENTED_EDGE ( 'NONE', *, *, #7728, .F. ) ;
#9685=VERTEX_POINT ( 'NONE', #10756 ) ;
#9726=CARTESIAN_POINT ( 'NONE',  ( 27.49999999999999645, 20.00000000000000355, 188.9999999999999716 ) ) ;
#9740=CARTESIAN_POINT ( 'NONE',  ( 1.000000000000000888, 20.00000000000000711, 170.9999999999999716 ) ) ;
#9746=CARTESIAN_POINT ( 'NONE',  ( 27.49999999999999645, 20.00000000000000355, 162.0000000000000000 ) ) ;
#9787=DIRECTION ( 'NONE',  ( -1.000000000000000000, 0.000000000000000000, 0.000000000000000000 ) ) ;
#9801=ORIENTED_EDGE ( 'NONE', *, *, #12257, .T. ) ;
#9805=CONICAL_SURFACE ( 'NONE', #1094, 25.50000000000000711, 0.7853981633974552734 ) ;
#9813=CARTESIAN_POINT ( 'NONE',  ( 27.49999999999999645, 20.00000000000000355, 197.9999999999999716 ) ) ;
#9816=AXIS2_PLACEMENT_3D ( 'NONE', #9418, #4587, #10415 ) ;
#9844=DIRECTION ( 'NONE',  ( -0.000000000000000000, -0.000000000000000000, 1.000000000000000000 ) ) ;
#9845=DIRECTION ( 'NONE',  ( 1.000000000000000000, 0.000000000000000000, 0.000000000000000000 ) ) ;
#9875=ORIENTED_EDGE ( 'NONE', *, *, #475, .T. ) ;
#9886=CARTESIAN_POINT ( 'NONE',  ( 4.000000000000000000, 20.00000000000000355, 189.9999999999999716 ) ) ;
#9932=PRODUCT_DEFINITION_CONTEXT ( 'detailed design', #8052, 'design' ) ;
#9955=CARTESIAN_POINT ( 'NONE',  ( 53.99999999999999289, 20.00000000000000711, 189.9999999999999716 ) ) ;
#10009=PRODUCT_DEFINITION_FORMATION_WITH_SPECIFIED_SOURCE ( 'ANY', '', #10963, .NOT_KNOWN. ) ;
#10013=SHAPE_REPRESENTATION ( 'Bearing', ( #9021 ), #2935 ) ;
#10029=EDGE_CURVE ( 'NONE', #6345, #4797, #9460, .T. ) ;
#10036=ORIENTED_EDGE ( 'NONE', *, *, #302, .F. ) ;
#10056=PRODUCT_DEFINITION_SHAPE ( 'NONE', 'NONE',  #10161 ) ;
#10095=ORIENTED_EDGE ( 'NONE', *, *, #10182, .T. ) ;
#10096=DIRECTION ( 'NONE',  ( 1.000000000000000000, 0.000000000000000000, 0.000000000000000000 ) ) ;
#10132=EDGE_CURVE ( 'NONE', #9159, #3577, #11488, .T. ) ;
#10161=PRODUCT_DEFINITION ( 'UNKNOWN', '', #10009, #9932 ) ;
#10182=EDGE_CURVE ( 'NONE', #9159, #11119, #9274, .T. ) ;
#10183=CARTESIAN_POINT ( 'NONE',  ( 1.000000000000000888, 20.00000000000000355, 189.0000000000000000 ) ) ;
#10210=EDGE_LOOP ( 'NONE', ( #4439, #8915, #3005, #2162 ) ) ;
#10237=EDGE_CURVE ( 'NONE', #4148, #8970, #151, .T. ) ;
#10245=EDGE_LOOP ( 'NONE', ( #3485, #3616, #1250, #8021 ) ) ;
#10286=VERTEX_POINT ( 'NONE', #9886 ) ;
#10361=ORIENTED_EDGE ( 'NONE', *, *, #7728, .T. ) ;
#10388=CIRCLE ( 'NONE', #870, 23.49999999999999289 ) ;
#10407=ORIENTED_EDGE ( 'NONE', *, *, #833, .T. ) ;
#10415=DIRECTION ( 'NONE',  ( 0.000000000000000000, 0.000000000000000000, -1.000000000000000000 ) ) ;
#10440=ORIENTED_EDGE ( 'NONE', *, *, #1553, .F. ) ;
#10461=DIRECTION ( 'NONE',  ( 0.000000000000000000, 0.000000000000000000, 1.000000000000000000 ) ) ;
#10492=DIRECTION ( 'NONE',  ( 0.7071067811865500152, 0.000000000000000000, 0.7071067811865451302 ) ) ;
#10505=EDGE_CURVE ( 'NONE', #5816, #10732, #4806, .T. ) ;
#10540=CARTESIAN_POINT ( 'NONE',  ( 52.99999999999998579, 20.00000000000000355, 169.9999999999999716 ) ) ;
#10541=DIRECTION ( 'NONE',  ( -0.000000000000000000, -1.000000000000000000, -0.000000000000000000 ) ) ;
#10572=EDGE_CURVE ( 'NONE', #3577, #10746, #8214, .T. ) ;
#10583=AXIS2_PLACEMENT_3D ( 'NONE', #6280, #386, #11038 ) ;
#10717=CARTESIAN_POINT ( 'NONE',  ( 27.49999999999999645, 20.00000000000000355, 170.9999999999999716 ) ) ;
#10721=( LENGTH_UNIT ( ) NAMED_UNIT ( * ) SI_UNIT ( .MILLI., .METRE. ) );
#10725=DIRECTION ( 'NONE',  ( 0.000000000000000000, 0.000000000000000000, 1.000000000000000000 ) ) ;
#10732=VERTEX_POINT ( 'NONE', #5705 ) ;
#10734=CARTESIAN_POINT ( 'NONE',  ( 1.999999999999988010, 20.00000000000000355, 189.9999999999999716 ) ) ;
#10735=ORIENTED_EDGE ( 'NONE', *, *, #1070, .T. ) ;
#10746=VERTEX_POINT ( 'NONE', #9634 ) ;
#10756=CARTESIAN_POINT ( 'NONE',  ( 44.99999999999996447, 20.00000000000000355, 172.0000000000000000 ) ) ;
#10817=VERTEX_POINT ( 'NONE', #10823 ) ;
#10818=AXIS2_PLACEMENT_3D ( 'NONE', #568, #631, #4374 ) ;
#10822=DIRECTION ( 'NONE',  ( 1.000000000000000000, 0.000000000000000000, 0.000000000000000000 ) ) ;
#10823=CARTESIAN_POINT ( 'NONE',  ( 53.99999999999999289, 20.00000000000000711, 189.0000000000000000 ) ) ;
#10883=DIRECTION ( 'NONE',  ( 0.000000000000000000, 0.000000000000000000, -1.000000000000000000 ) ) ;
#10889=DIRECTION ( 'NONE',  ( -1.000000000000000000, 0.000000000000000000, 0.000000000000000000 ) ) ;
#10926=DIRECTION ( 'NONE',  ( 1.000000000000000000, 0.000000000000000000, 0.000000000000000000 ) ) ;
#10940=DIRECTION ( 'NONE',  ( -0.000000000000000000, -0.000000000000000000, -1.000000000000000000 ) ) ;
#10963=PRODUCT ( 'Bearing', 'Bearing', '', ( #953 ) ) ;
#10986=VERTEX_POINT ( 'NONE', #7525 ) ;
#11038=DIRECTION ( 'NONE',  ( 1.000000000000000000, 0.000000000000000000, 0.000000000000000000 ) ) ;
#11061=DIRECTION ( 'NONE',  ( 1.000000000000000000, 0.000000000000000000, 0.000000000000000000 ) ) ;
#11116=ORIENTED_EDGE ( 'NONE', *, *, #7153, .T. ) ;
#11119=VERTEX_POINT ( 'NONE', #12346 ) ;
#11121=DIRECTION ( 'NONE',  ( 1.000000000000000000, 0.000000000000000000, 0.000000000000000000 ) ) ;
#11187=CYLINDRICAL_SURFACE ( 'NONE', #8105, 26.49999999999999645 ) ;
#11188=CYLINDRICAL_SURFACE ( 'NONE', #11702, 26.49999999999999645 ) ;
#11227=VECTOR ( 'NONE', #182, 1000.000000000000000 ) ;
#11236=ORIENTED_EDGE ( 'NONE', *, *, #8321, .T. ) ;
#11244=PLANE ( 'NONE',  #6173 ) ;
#11246=CARTESIAN_POINT ( 'NONE',  ( 36.99999999999999289, 20.00000000000000355, 171.0000000000000000 ) ) ;
#11267=CIRCLE ( 'NONE', #3168, 10.00000000000000178 ) ;
#11273=DIRECTION ( 'NONE',  ( 0.000000000000000000, -1.000000000000000000, 0.000000000000000000 ) ) ;
#11328=EDGE_CURVE ( 'NONE', #10732, #5816, #7586, .T. ) ;
#11340=CARTESIAN_POINT ( 'NONE',  ( 44.99999999999996447, 20.00000000000000355, 162.0000000000000000 ) ) ;
#11345=CONICAL_SURFACE ( 'NONE', #2634, 26.49999999999999645, 0.7853981633974517207 ) ;
#11363=CIRCLE ( 'NONE', #5897, 25.49999999999998934 ) ;
#11378=EDGE_CURVE ( 'NONE', #3577, #9159, #1700, .T. ) ;
#11386=EDGE_LOOP ( 'NONE', ( #3901, #6792, #10036, #3458 ) ) ;
#11409=AXIS2_PLACEMENT_3D ( 'NONE', #3143, #11651, #2959 ) ;
#11433=CARTESIAN_POINT ( 'NONE',  ( 0.000000000000000000, 0.000000000000000000, 0.000000000000000000 ) ) ;
#11488=CIRCLE ( 'NONE', #1369, 9.499999999999994671 ) ;
#11489=ORIENTED_EDGE ( 'NONE', *, *, #10572, .F. ) ;
#11491=ORIENTED_EDGE ( 'NONE', *, *, #3025, .F. ) ;
#11534=CYLINDRICAL_SURFACE ( 'NONE', #7787, 7.500000000000000000 ) ;
#11567=ORIENTED_EDGE ( 'NONE', *, *, #6998, .F. ) ;
#11578=DIRECTION ( 'NONE',  ( 1.000000000000000000, 0.000000000000000000, 0.000000000000000000 ) ) ;
#11607=CIRCLE ( 'NONE', #2075, 17.49999999999996803 ) ;
#11623=DIRECTION ( 'NONE',  ( -0.000000000000000000, -0.000000000000000000, -1.000000000000000000 ) ) ;
#11633=ORIENTED_EDGE ( 'NONE', *, *, #5095, .F. ) ;
#11641=DIRECTION ( 'NONE',  ( -0.7071067811865500152, 8.659560562354962440E-17, 0.7071067811865451302 ) ) ;
#11651=DIRECTION ( 'NONE',  ( 0.000000000000000000, 0.000000000000000000, -1.000000000000000000 ) ) ;
#11655=UNCERTAINTY_MEASURE_WITH_UNIT (LENGTH_MEASURE( 1.000000000000000082E-05 ), #362, 'distance_accuracy_value', 'NONE');
#11665=DIRECTION ( 'NONE',  ( 1.000000000000000000, 0.000000000000000000, -0.000000000000000000 ) ) ;
#11687=CYLINDRICAL_SURFACE ( 'NONE', #3571, 7.500000000000000000 ) ;
#11702=AXIS2_PLACEMENT_3D ( 'NONE', #6309, #9230, #12018 ) ;
#11720=ADVANCED_FACE ( 'NONE', ( #6341 ), #3721, .F. ) ;
#11728=CARTESIAN_POINT ( 'NONE',  ( 27.49999999999999645, 20.00000000000000355, 189.9999999999999716 ) ) ;
#11748=DIRECTION ( 'NONE',  ( 0.7071067811865524577, 8.659560562354993255E-17, -0.7071067811865426878 ) ) ;
#11803=DIRECTION ( 'NONE',  ( 1.000000000000000000, 0.000000000000000000, 0.000000000000000000 ) ) ;
#11824=DIRECTION ( 'NONE',  ( 0.000000000000000000, 0.000000000000000000, 1.000000000000000000 ) ) ;
#11839=ORIENTED_EDGE ( 'NONE', *, *, #9611, .F. ) ;
#11843=AXIS2_PLACEMENT_3D ( 'NONE', #12332, #12394, #783 ) ;
#11846=ADVANCED_FACE ( 'NONE', ( #1821 ), #11534, .F. ) ;
#11898=AXIS2_PLACEMENT_3D ( 'NONE', #12480, #8426, #12296 ) ;
#11947=ADVANCED_FACE ( 'NONE', ( #9573, #8740 ), #3917, .T. ) ;
#11960=EDGE_CURVE ( 'NONE', #2177, #4738, #1702, .T. ) ;
#11985=CIRCLE ( 'NONE', #9145, 26.49999999999999645 ) ;
#11998=ORIENTED_EDGE ( 'NONE', *, *, #10029, .T. ) ;
#12009=ORIENTED_EDGE ( 'NONE', *, *, #7622, .F. ) ;
#12018=DIRECTION ( 'NONE',  ( -1.000000000000000000, 0.000000000000000000, 0.000000000000000000 ) ) ;
#12033=EDGE_CURVE ( 'NONE', #2177, #4576, #2926, .T. ) ;
#12034=TOROIDAL_SURFACE ( 'NONE', #6551, 17.50000000000000355, 10.00000000000000000 ) ;
#12096=AXIS2_PLACEMENT_3D ( 'NONE', #5633, #2965, #2902 ) ;
#12124=ORIENTED_EDGE ( 'NONE', *, *, #3025, .T. ) ;
#12213=( NAMED_UNIT ( * ) PLANE_ANGLE_UNIT ( ) SI_UNIT ( $, .RADIAN. ) );
#12217=CARTESIAN_POINT ( 'NONE',  ( 9.999999999999991118, 20.00000000000000355, 197.9999999999999716 ) ) ;
#12257=EDGE_CURVE ( 'NONE', #9626, #1347, #5373, .T. ) ;
#12296=DIRECTION ( 'NONE',  ( 1.000000000000000000, 0.000000000000000000, 0.000000000000000000 ) ) ;
#12301=FACE_OUTER_BOUND ( 'NONE', #10245, .T. ) ;
#12304=DIRECTION ( 'NONE',  ( -1.000000000000000000, 0.000000000000000000, 0.000000000000000000 ) ) ;
#12332=CARTESIAN_POINT ( 'NONE',  ( 27.49999999999999645, 20.00000000000000355, 171.0000000000000000 ) ) ;
#12345=LINE ( 'NONE', #6502, #3712 ) ;
#12346=CARTESIAN_POINT ( 'NONE',  ( 41.35889894354065177, 20.00000000000000355, 172.0000000000000000 ) ) ;
#12378=AXIS2_PLACEMENT_3D ( 'NONE', #1349, #4316, #10096 ) ;
#12380=ADVANCED_FACE ( 'NONE', ( #1193, #3381 ), #11244, .T. ) ;
#12382=EDGE_LOOP ( 'NONE', ( #8303, #7164 ) ) ;
#12387=ORIENTED_EDGE ( 'NONE', *, *, #3620, .T. ) ;
#12394=DIRECTION ( 'NONE',  ( -0.000000000000000000, -0.000000000000000000, 1.000000000000000000 ) ) ;
#12429=DIRECTION ( 'NONE',  ( 0.000000000000000000, 0.000000000000000000, 1.000000000000000000 ) ) ;
#12480=CARTESIAN_POINT ( 'NONE',  ( 27.49999999999999645, 20.00000000000000355, 187.9999999999999716 ) ) ;
#12487=DIRECTION ( 'NONE',  ( 1.000000000000000000, 0.000000000000000000, 0.000000000000000000 ) ) ;
#12513=CARTESIAN_POINT ( 'NONE',  ( 27.49999999999999645, 20.00000000000000355, 187.9999999999999716 ) ) ;
#12514=AXIS2_PLACEMENT_3D ( 'NONE', #6986, #11623, #6918 ) ;
#12527=CARTESIAN_POINT ( 'NONE',  ( 27.49999999999999645, 20.00000000000000355, 189.0000000000000000 ) ) ;
#12533=DIRECTION ( 'NONE',  ( -0.000000000000000000, -0.000000000000000000, 1.000000000000000000 ) ) ;
#12578=COLOUR_RGB('Grey',0.48,0.52,0.57);
#12579=FILL_AREA_STYLE_COLOUR('',#12578);
#12580=FILL_AREA_STYLE('',(#12579));
#12581=SURFACE_STYLE_FILL_AREA(#12580);
#12582=SURFACE_SIDE_STYLE('',(#12581));
#12583=SURFACE_STYLE_USAGE(.BOTH.,#12582);
#12584=PRESENTATION_STYLE_ASSIGNMENT((#12583));
ENDSEC;
END-ISO-10303-21;
